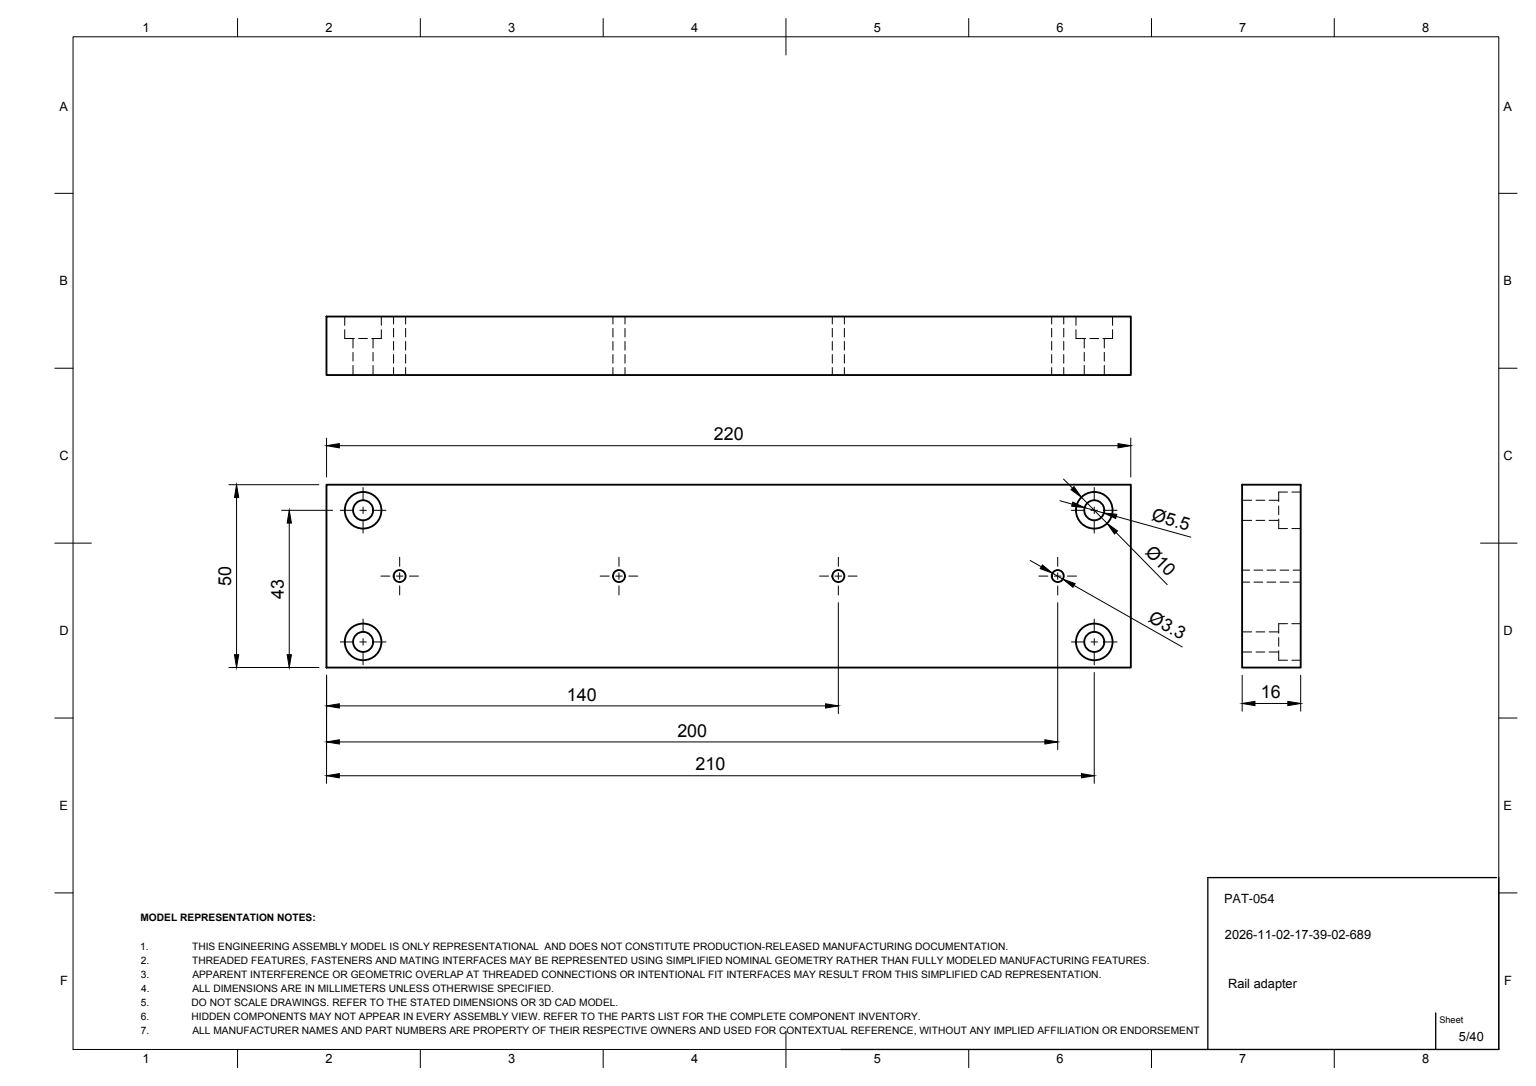
ISO-10303-21;
HEADER;
/* Generated by software containing ST-Developer
 * from STEP Tools, Inc. (www.steptools.com) 
 */

FILE_DESCRIPTION(
/* description */ ('PAT-054'),
/* implementation_level */ '2;1');

FILE_NAME(
/* name */ 'Rail adapter.step',
/* time_stamp */ '2026-10-29T16:38:13-07:00',
/* author */ (''),
/* organization */ (''),
/* preprocessor_version */ 'ST-DEVELOPER v20.2',
/* originating_system */ 'Autodesk Translation Framework v15.17.0.0',
/* authorisation */ '');

FILE_SCHEMA (('AUTOMOTIVE_DESIGN { 1 0 10303 214 3 1 1 }'));
ENDSEC;

DATA;
#10=MECHANICAL_DESIGN_GEOMETRIC_PRESENTATION_REPRESENTATION('',(#900),#33981);
#812=SHAPE_REPRESENTATION_RELATIONSHIP('SRR','None',#34185,#856);
#856=ADVANCED_BREP_SHAPE_REPRESENTATION('',(#959),#33933);
#900=STYLED_ITEM('',(#34510),#959);
#959=MANIFOLD_SOLID_BREP('Body1',#13011);
#1044=FACE_BOUND('',#2358,.T.);
#1045=FACE_BOUND('',#2361,.T.);
#1046=FACE_BOUND('',#2364,.T.);
#1047=FACE_BOUND('',#2367,.T.);
#1048=FACE_BOUND('',#2377,.T.);
#1049=FACE_BOUND('',#2378,.T.);
#1050=FACE_BOUND('',#2379,.T.);
#1051=FACE_BOUND('',#2380,.T.);
#1052=FACE_BOUND('',#2381,.T.);
#1053=FACE_BOUND('',#2382,.T.);
#1054=FACE_BOUND('',#2383,.T.);
#1055=FACE_BOUND('',#2384,.T.);
#1056=FACE_BOUND('',#2386,.T.);
#1057=FACE_BOUND('',#2387,.T.);
#1058=FACE_BOUND('',#2388,.T.);
#1059=FACE_BOUND('',#2389,.T.);
#1060=FACE_BOUND('',#2390,.T.);
#1061=FACE_BOUND('',#2391,.T.);
#1062=FACE_BOUND('',#2392,.T.);
#1063=FACE_BOUND('',#2393,.T.);
#1234=PLANE('',#13632);
#1235=PLANE('',#13637);
#1236=PLANE('',#13642);
#1237=PLANE('',#13647);
#1238=PLANE('',#13657);
#1239=PLANE('',#13658);
#1240=PLANE('',#13659);
#1241=PLANE('',#13660);
#1242=PLANE('',#13661);
#1243=PLANE('',#13662);
#1597=FACE_OUTER_BOUND('',#2352,.T.);
#1598=FACE_OUTER_BOUND('',#2353,.T.);
#1599=FACE_OUTER_BOUND('',#2354,.T.);
#1600=FACE_OUTER_BOUND('',#2355,.T.);
#1601=FACE_OUTER_BOUND('',#2356,.T.);
#1602=FACE_OUTER_BOUND('',#2357,.T.);
#1603=FACE_OUTER_BOUND('',#2359,.T.);
#1604=FACE_OUTER_BOUND('',#2360,.T.);
#1605=FACE_OUTER_BOUND('',#2362,.T.);
#1606=FACE_OUTER_BOUND('',#2363,.T.);
#1607=FACE_OUTER_BOUND('',#2365,.T.);
#1608=FACE_OUTER_BOUND('',#2366,.T.);
#1609=FACE_OUTER_BOUND('',#2368,.T.);
#1610=FACE_OUTER_BOUND('',#2369,.T.);
#1611=FACE_OUTER_BOUND('',#2370,.T.);
#1612=FACE_OUTER_BOUND('',#2371,.T.);
#1613=FACE_OUTER_BOUND('',#2372,.T.);
#1614=FACE_OUTER_BOUND('',#2373,.T.);
#1615=FACE_OUTER_BOUND('',#2374,.T.);
#1616=FACE_OUTER_BOUND('',#2375,.T.);
#1617=FACE_OUTER_BOUND('',#2376,.T.);
#1618=FACE_OUTER_BOUND('',#2385,.T.);
#2352=EDGE_LOOP('',(#8609,#8610,#8611,#8612));
#2353=EDGE_LOOP('',(#8613,#8614,#8615,#8616));
#2354=EDGE_LOOP('',(#8617,#8618,#8619,#8620));
#2355=EDGE_LOOP('',(#8621,#8622,#8623,#8624));
#2356=EDGE_LOOP('',(#8625,#8626,#8627,#8628));
#2357=EDGE_LOOP('',(#8629));
#2358=EDGE_LOOP('',(#8630));
#2359=EDGE_LOOP('',(#8631,#8632,#8633,#8634));
#2360=EDGE_LOOP('',(#8635));
#2361=EDGE_LOOP('',(#8636));
#2362=EDGE_LOOP('',(#8637,#8638,#8639,#8640));
#2363=EDGE_LOOP('',(#8641));
#2364=EDGE_LOOP('',(#8642));
#2365=EDGE_LOOP('',(#8643,#8644,#8645,#8646));
#2366=EDGE_LOOP('',(#8647));
#2367=EDGE_LOOP('',(#8648));
#2368=EDGE_LOOP('',(#8649,#8650,#8651,#8652));
#2369=EDGE_LOOP('',(#8653,#8654,#8655,#8656));
#2370=EDGE_LOOP('',(#8657,#8658,#8659,#8660));
#2371=EDGE_LOOP('',(#8661,#8662,#8663,#8664));
#2372=EDGE_LOOP('',(#8665,#8666,#8667,#8668));
#2373=EDGE_LOOP('',(#8669,#8670,#8671,#8672));
#2374=EDGE_LOOP('',(#8673,#8674,#8675,#8676));
#2375=EDGE_LOOP('',(#8677,#8678,#8679,#8680));
#2376=EDGE_LOOP('',(#8681,#8682,#8683,#8684));
#2377=EDGE_LOOP('',(#8685));
#2378=EDGE_LOOP('',(#8686));
#2379=EDGE_LOOP('',(#8687));
#2380=EDGE_LOOP('',(#8688));
#2381=EDGE_LOOP('',(#8689));
#2382=EDGE_LOOP('',(#8690));
#2383=EDGE_LOOP('',(#8691));
#2384=EDGE_LOOP('',(#8692));
#2385=EDGE_LOOP('',(#8693,#8694,#8695,#8696));
#2386=EDGE_LOOP('',(#8697));
#2387=EDGE_LOOP('',(#8698));
#2388=EDGE_LOOP('',(#8699));
#2389=EDGE_LOOP('',(#8700));
#2390=EDGE_LOOP('',(#8701));
#2391=EDGE_LOOP('',(#8702));
#2392=EDGE_LOOP('',(#8703));
#2393=EDGE_LOOP('',(#8704));
#3265=LINE('',#18616,#4199);
#3266=LINE('',#18622,#4200);
#3267=LINE('',#18628,#4201);
#3268=LINE('',#18634,#4202);
#3269=LINE('',#18640,#4203);
#3270=LINE('',#18649,#4204);
#3271=LINE('',#18658,#4205);
#3272=LINE('',#18667,#4206);
#3273=LINE('',#18675,#4207);
#3274=LINE('',#18679,#4208);
#3275=LINE('',#18683,#4209);
#3276=LINE('',#18687,#4210);
#3277=LINE('',#18691,#4211);
#3278=LINE('',#18693,#4212);
#3279=LINE('',#18695,#4213);
#3280=LINE('',#18696,#4214);
#3281=LINE('',#18699,#4215);
#3282=LINE('',#18701,#4216);
#3283=LINE('',#18702,#4217);
#3284=LINE('',#18705,#4218);
#3285=LINE('',#18707,#4219);
#3286=LINE('',#18708,#4220);
#3287=LINE('',#18710,#4221);
#3288=LINE('',#18711,#4222);
#4199=VECTOR('',#15038,0.164999999999999);
#4200=VECTOR('',#15045,0.164999999999999);
#4201=VECTOR('',#15052,0.165);
#4202=VECTOR('',#15059,0.164999999999999);
#4203=VECTOR('',#15066,0.5);
#4204=VECTOR('',#15077,0.5);
#4205=VECTOR('',#15088,0.5);
#4206=VECTOR('',#15099,0.5);
#4207=VECTOR('',#15110,0.274999999999999);
#4208=VECTOR('',#15115,0.275);
#4209=VECTOR('',#15120,0.275);
#4210=VECTOR('',#15125,0.274999999999999);
#4211=VECTOR('',#15128,1.);
#4212=VECTOR('',#15129,1.);
#4213=VECTOR('',#15130,1.);
#4214=VECTOR('',#15131,1.);
#4215=VECTOR('',#15134,1.);
#4216=VECTOR('',#15135,1.);
#4217=VECTOR('',#15136,1.);
#4218=VECTOR('',#15139,1.);
#4219=VECTOR('',#15140,1.);
#4220=VECTOR('',#15141,1.);
#4221=VECTOR('',#15144,1.);
#4222=VECTOR('',#15145,1.);
#5137=CIRCLE('',#13618,0.164999999999999);
#5138=CIRCLE('',#13619,0.164999999999999);
#5139=CIRCLE('',#13621,0.164999999999999);
#5140=CIRCLE('',#13622,0.164999999999999);
#5141=CIRCLE('',#13624,0.165);
#5142=CIRCLE('',#13625,0.165);
#5143=CIRCLE('',#13627,0.164999999999999);
#5144=CIRCLE('',#13628,0.164999999999999);
#5145=CIRCLE('',#13630,0.5);
#5146=CIRCLE('',#13631,0.5);
#5147=CIRCLE('',#13633,0.274999999999999);
#5148=CIRCLE('',#13635,0.5);
#5149=CIRCLE('',#13636,0.5);
#5150=CIRCLE('',#13638,0.275);
#5151=CIRCLE('',#13640,0.5);
#5152=CIRCLE('',#13641,0.5);
#5153=CIRCLE('',#13643,0.275);
#5154=CIRCLE('',#13645,0.5);
#5155=CIRCLE('',#13646,0.5);
#5156=CIRCLE('',#13648,0.274999999999999);
#5157=CIRCLE('',#13650,0.274999999999999);
#5158=CIRCLE('',#13652,0.275);
#5159=CIRCLE('',#13654,0.275);
#5160=CIRCLE('',#13656,0.274999999999999);
#5610=VERTEX_POINT('',#18613);
#5611=VERTEX_POINT('',#18615);
#5612=VERTEX_POINT('',#18619);
#5613=VERTEX_POINT('',#18621);
#5614=VERTEX_POINT('',#18625);
#5615=VERTEX_POINT('',#18627);
#5616=VERTEX_POINT('',#18631);
#5617=VERTEX_POINT('',#18633);
#5618=VERTEX_POINT('',#18637);
#5619=VERTEX_POINT('',#18639);
#5620=VERTEX_POINT('',#18643);
#5621=VERTEX_POINT('',#18646);
#5622=VERTEX_POINT('',#18648);
#5623=VERTEX_POINT('',#18652);
#5624=VERTEX_POINT('',#18655);
#5625=VERTEX_POINT('',#18657);
#5626=VERTEX_POINT('',#18661);
#5627=VERTEX_POINT('',#18664);
#5628=VERTEX_POINT('',#18666);
#5629=VERTEX_POINT('',#18670);
#5630=VERTEX_POINT('',#18673);
#5631=VERTEX_POINT('',#18677);
#5632=VERTEX_POINT('',#18681);
#5633=VERTEX_POINT('',#18685);
#5634=VERTEX_POINT('',#18689);
#5635=VERTEX_POINT('',#18690);
#5636=VERTEX_POINT('',#18692);
#5637=VERTEX_POINT('',#18694);
#5638=VERTEX_POINT('',#18698);
#5639=VERTEX_POINT('',#18700);
#5640=VERTEX_POINT('',#18704);
#5641=VERTEX_POINT('',#18706);
#6804=EDGE_CURVE('',#5610,#5610,#5137,.T.);
#6805=EDGE_CURVE('',#5610,#5611,#3265,.T.);
#6806=EDGE_CURVE('',#5611,#5611,#5138,.T.);
#6807=EDGE_CURVE('',#5612,#5612,#5139,.T.);
#6808=EDGE_CURVE('',#5612,#5613,#3266,.T.);
#6809=EDGE_CURVE('',#5613,#5613,#5140,.T.);
#6810=EDGE_CURVE('',#5614,#5614,#5141,.T.);
#6811=EDGE_CURVE('',#5614,#5615,#3267,.T.);
#6812=EDGE_CURVE('',#5615,#5615,#5142,.T.);
#6813=EDGE_CURVE('',#5616,#5616,#5143,.T.);
#6814=EDGE_CURVE('',#5616,#5617,#3268,.T.);
#6815=EDGE_CURVE('',#5617,#5617,#5144,.T.);
#6816=EDGE_CURVE('',#5618,#5618,#5145,.T.);
#6817=EDGE_CURVE('',#5618,#5619,#3269,.T.);
#6818=EDGE_CURVE('',#5619,#5619,#5146,.T.);
#6819=EDGE_CURVE('',#5620,#5620,#5147,.T.);
#6820=EDGE_CURVE('',#5621,#5621,#5148,.T.);
#6821=EDGE_CURVE('',#5621,#5622,#3270,.T.);
#6822=EDGE_CURVE('',#5622,#5622,#5149,.T.);
#6823=EDGE_CURVE('',#5623,#5623,#5150,.T.);
#6824=EDGE_CURVE('',#5624,#5624,#5151,.T.);
#6825=EDGE_CURVE('',#5624,#5625,#3271,.T.);
#6826=EDGE_CURVE('',#5625,#5625,#5152,.T.);
#6827=EDGE_CURVE('',#5626,#5626,#5153,.T.);
#6828=EDGE_CURVE('',#5627,#5627,#5154,.T.);
#6829=EDGE_CURVE('',#5627,#5628,#3272,.T.);
#6830=EDGE_CURVE('',#5628,#5628,#5155,.T.);
#6831=EDGE_CURVE('',#5629,#5629,#5156,.T.);
#6832=EDGE_CURVE('',#5630,#5630,#5157,.T.);
#6833=EDGE_CURVE('',#5630,#5620,#3273,.T.);
#6834=EDGE_CURVE('',#5631,#5631,#5158,.T.);
#6835=EDGE_CURVE('',#5631,#5623,#3274,.T.);
#6836=EDGE_CURVE('',#5632,#5632,#5159,.T.);
#6837=EDGE_CURVE('',#5632,#5626,#3275,.T.);
#6838=EDGE_CURVE('',#5633,#5633,#5160,.T.);
#6839=EDGE_CURVE('',#5633,#5629,#3276,.T.);
#6840=EDGE_CURVE('',#5634,#5635,#3277,.T.);
#6841=EDGE_CURVE('',#5635,#5636,#3278,.T.);
#6842=EDGE_CURVE('',#5637,#5636,#3279,.T.);
#6843=EDGE_CURVE('',#5634,#5637,#3280,.T.);
#6844=EDGE_CURVE('',#5638,#5634,#3281,.T.);
#6845=EDGE_CURVE('',#5639,#5637,#3282,.T.);
#6846=EDGE_CURVE('',#5638,#5639,#3283,.T.);
#6847=EDGE_CURVE('',#5640,#5638,#3284,.T.);
#6848=EDGE_CURVE('',#5641,#5639,#3285,.T.);
#6849=EDGE_CURVE('',#5640,#5641,#3286,.T.);
#6850=EDGE_CURVE('',#5635,#5640,#3287,.T.);
#6851=EDGE_CURVE('',#5636,#5641,#3288,.T.);
#8609=ORIENTED_EDGE('',*,*,#6804,.F.);
#8610=ORIENTED_EDGE('',*,*,#6805,.T.);
#8611=ORIENTED_EDGE('',*,*,#6806,.F.);
#8612=ORIENTED_EDGE('',*,*,#6805,.F.);
#8613=ORIENTED_EDGE('',*,*,#6807,.F.);
#8614=ORIENTED_EDGE('',*,*,#6808,.T.);
#8615=ORIENTED_EDGE('',*,*,#6809,.F.);
#8616=ORIENTED_EDGE('',*,*,#6808,.F.);
#8617=ORIENTED_EDGE('',*,*,#6810,.F.);
#8618=ORIENTED_EDGE('',*,*,#6811,.T.);
#8619=ORIENTED_EDGE('',*,*,#6812,.F.);
#8620=ORIENTED_EDGE('',*,*,#6811,.F.);
#8621=ORIENTED_EDGE('',*,*,#6813,.F.);
#8622=ORIENTED_EDGE('',*,*,#6814,.T.);
#8623=ORIENTED_EDGE('',*,*,#6815,.F.);
#8624=ORIENTED_EDGE('',*,*,#6814,.F.);
#8625=ORIENTED_EDGE('',*,*,#6816,.F.);
#8626=ORIENTED_EDGE('',*,*,#6817,.T.);
#8627=ORIENTED_EDGE('',*,*,#6818,.F.);
#8628=ORIENTED_EDGE('',*,*,#6817,.F.);
#8629=ORIENTED_EDGE('',*,*,#6816,.T.);
#8630=ORIENTED_EDGE('',*,*,#6819,.F.);
#8631=ORIENTED_EDGE('',*,*,#6820,.F.);
#8632=ORIENTED_EDGE('',*,*,#6821,.T.);
#8633=ORIENTED_EDGE('',*,*,#6822,.F.);
#8634=ORIENTED_EDGE('',*,*,#6821,.F.);
#8635=ORIENTED_EDGE('',*,*,#6820,.T.);
#8636=ORIENTED_EDGE('',*,*,#6823,.F.);
#8637=ORIENTED_EDGE('',*,*,#6824,.F.);
#8638=ORIENTED_EDGE('',*,*,#6825,.T.);
#8639=ORIENTED_EDGE('',*,*,#6826,.F.);
#8640=ORIENTED_EDGE('',*,*,#6825,.F.);
#8641=ORIENTED_EDGE('',*,*,#6824,.T.);
#8642=ORIENTED_EDGE('',*,*,#6827,.F.);
#8643=ORIENTED_EDGE('',*,*,#6828,.F.);
#8644=ORIENTED_EDGE('',*,*,#6829,.T.);
#8645=ORIENTED_EDGE('',*,*,#6830,.F.);
#8646=ORIENTED_EDGE('',*,*,#6829,.F.);
#8647=ORIENTED_EDGE('',*,*,#6828,.T.);
#8648=ORIENTED_EDGE('',*,*,#6831,.F.);
#8649=ORIENTED_EDGE('',*,*,#6832,.F.);
#8650=ORIENTED_EDGE('',*,*,#6833,.T.);
#8651=ORIENTED_EDGE('',*,*,#6819,.T.);
#8652=ORIENTED_EDGE('',*,*,#6833,.F.);
#8653=ORIENTED_EDGE('',*,*,#6834,.F.);
#8654=ORIENTED_EDGE('',*,*,#6835,.T.);
#8655=ORIENTED_EDGE('',*,*,#6823,.T.);
#8656=ORIENTED_EDGE('',*,*,#6835,.F.);
#8657=ORIENTED_EDGE('',*,*,#6836,.F.);
#8658=ORIENTED_EDGE('',*,*,#6837,.T.);
#8659=ORIENTED_EDGE('',*,*,#6827,.T.);
#8660=ORIENTED_EDGE('',*,*,#6837,.F.);
#8661=ORIENTED_EDGE('',*,*,#6838,.F.);
#8662=ORIENTED_EDGE('',*,*,#6839,.T.);
#8663=ORIENTED_EDGE('',*,*,#6831,.T.);
#8664=ORIENTED_EDGE('',*,*,#6839,.F.);
#8665=ORIENTED_EDGE('',*,*,#6840,.T.);
#8666=ORIENTED_EDGE('',*,*,#6841,.T.);
#8667=ORIENTED_EDGE('',*,*,#6842,.F.);
#8668=ORIENTED_EDGE('',*,*,#6843,.F.);
#8669=ORIENTED_EDGE('',*,*,#6844,.T.);
#8670=ORIENTED_EDGE('',*,*,#6843,.T.);
#8671=ORIENTED_EDGE('',*,*,#6845,.F.);
#8672=ORIENTED_EDGE('',*,*,#6846,.F.);
#8673=ORIENTED_EDGE('',*,*,#6847,.T.);
#8674=ORIENTED_EDGE('',*,*,#6846,.T.);
#8675=ORIENTED_EDGE('',*,*,#6848,.F.);
#8676=ORIENTED_EDGE('',*,*,#6849,.F.);
#8677=ORIENTED_EDGE('',*,*,#6850,.T.);
#8678=ORIENTED_EDGE('',*,*,#6849,.T.);
#8679=ORIENTED_EDGE('',*,*,#6851,.F.);
#8680=ORIENTED_EDGE('',*,*,#6841,.F.);
#8681=ORIENTED_EDGE('',*,*,#6851,.T.);
#8682=ORIENTED_EDGE('',*,*,#6848,.T.);
#8683=ORIENTED_EDGE('',*,*,#6845,.T.);
#8684=ORIENTED_EDGE('',*,*,#6842,.T.);
#8685=ORIENTED_EDGE('',*,*,#6818,.T.);
#8686=ORIENTED_EDGE('',*,*,#6822,.T.);
#8687=ORIENTED_EDGE('',*,*,#6826,.T.);
#8688=ORIENTED_EDGE('',*,*,#6830,.T.);
#8689=ORIENTED_EDGE('',*,*,#6815,.T.);
#8690=ORIENTED_EDGE('',*,*,#6812,.T.);
#8691=ORIENTED_EDGE('',*,*,#6809,.T.);
#8692=ORIENTED_EDGE('',*,*,#6806,.T.);
#8693=ORIENTED_EDGE('',*,*,#6850,.F.);
#8694=ORIENTED_EDGE('',*,*,#6840,.F.);
#8695=ORIENTED_EDGE('',*,*,#6844,.F.);
#8696=ORIENTED_EDGE('',*,*,#6847,.F.);
#8697=ORIENTED_EDGE('',*,*,#6838,.T.);
#8698=ORIENTED_EDGE('',*,*,#6836,.T.);
#8699=ORIENTED_EDGE('',*,*,#6834,.T.);
#8700=ORIENTED_EDGE('',*,*,#6832,.T.);
#8701=ORIENTED_EDGE('',*,*,#6813,.T.);
#8702=ORIENTED_EDGE('',*,*,#6810,.T.);
#8703=ORIENTED_EDGE('',*,*,#6807,.T.);
#8704=ORIENTED_EDGE('',*,*,#6804,.T.);
#11995=CYLINDRICAL_SURFACE('',#13617,0.164999999999999);
#11996=CYLINDRICAL_SURFACE('',#13620,0.164999999999999);
#11997=CYLINDRICAL_SURFACE('',#13623,0.165);
#11998=CYLINDRICAL_SURFACE('',#13626,0.164999999999999);
#11999=CYLINDRICAL_SURFACE('',#13629,0.5);
#12000=CYLINDRICAL_SURFACE('',#13634,0.5);
#12001=CYLINDRICAL_SURFACE('',#13639,0.5);
#12002=CYLINDRICAL_SURFACE('',#13644,0.5);
#12003=CYLINDRICAL_SURFACE('',#13649,0.274999999999999);
#12004=CYLINDRICAL_SURFACE('',#13651,0.275);
#12005=CYLINDRICAL_SURFACE('',#13653,0.275);
#12006=CYLINDRICAL_SURFACE('',#13655,0.274999999999999);
#12309=ADVANCED_FACE('',(#1597),#11995,.F.);
#12310=ADVANCED_FACE('',(#1598),#11996,.F.);
#12311=ADVANCED_FACE('',(#1599),#11997,.F.);
#12312=ADVANCED_FACE('',(#1600),#11998,.F.);
#12313=ADVANCED_FACE('',(#1601),#11999,.F.);
#12314=ADVANCED_FACE('',(#1602,#1044),#1234,.T.);
#12315=ADVANCED_FACE('',(#1603),#12000,.F.);
#12316=ADVANCED_FACE('',(#1604,#1045),#1235,.T.);
#12317=ADVANCED_FACE('',(#1605),#12001,.F.);
#12318=ADVANCED_FACE('',(#1606,#1046),#1236,.T.);
#12319=ADVANCED_FACE('',(#1607),#12002,.F.);
#12320=ADVANCED_FACE('',(#1608,#1047),#1237,.T.);
#12321=ADVANCED_FACE('',(#1609),#12003,.F.);
#12322=ADVANCED_FACE('',(#1610),#12004,.F.);
#12323=ADVANCED_FACE('',(#1611),#12005,.F.);
#12324=ADVANCED_FACE('',(#1612),#12006,.F.);
#12325=ADVANCED_FACE('',(#1613),#1238,.T.);
#12326=ADVANCED_FACE('',(#1614),#1239,.T.);
#12327=ADVANCED_FACE('',(#1615),#1240,.T.);
#12328=ADVANCED_FACE('',(#1616),#1241,.T.);
#12329=ADVANCED_FACE('',(#1617,#1048,#1049,#1050,#1051,#1052,#1053,#1054,
#1055),#1242,.T.);
#12330=ADVANCED_FACE('',(#1618,#1056,#1057,#1058,#1059,#1060,#1061,#1062,
#1063),#1243,.F.);
#13011=CLOSED_SHELL('',(#12309,#12310,#12311,#12312,#12313,#12314,#12315,
#12316,#12317,#12318,#12319,#12320,#12321,#12322,#12323,#12324,#12325,#12326,
#12327,#12328,#12329,#12330));
#13616=AXIS2_PLACEMENT_3D('',#18611,#15032,#15033);
#13617=AXIS2_PLACEMENT_3D('',#18612,#15034,#15035);
#13618=AXIS2_PLACEMENT_3D('',#18614,#15036,#15037);
#13619=AXIS2_PLACEMENT_3D('',#18617,#15039,#15040);
#13620=AXIS2_PLACEMENT_3D('',#18618,#15041,#15042);
#13621=AXIS2_PLACEMENT_3D('',#18620,#15043,#15044);
#13622=AXIS2_PLACEMENT_3D('',#18623,#15046,#15047);
#13623=AXIS2_PLACEMENT_3D('',#18624,#15048,#15049);
#13624=AXIS2_PLACEMENT_3D('',#18626,#15050,#15051);
#13625=AXIS2_PLACEMENT_3D('',#18629,#15053,#15054);
#13626=AXIS2_PLACEMENT_3D('',#18630,#15055,#15056);
#13627=AXIS2_PLACEMENT_3D('',#18632,#15057,#15058);
#13628=AXIS2_PLACEMENT_3D('',#18635,#15060,#15061);
#13629=AXIS2_PLACEMENT_3D('',#18636,#15062,#15063);
#13630=AXIS2_PLACEMENT_3D('',#18638,#15064,#15065);
#13631=AXIS2_PLACEMENT_3D('',#18641,#15067,#15068);
#13632=AXIS2_PLACEMENT_3D('',#18642,#15069,#15070);
#13633=AXIS2_PLACEMENT_3D('',#18644,#15071,#15072);
#13634=AXIS2_PLACEMENT_3D('',#18645,#15073,#15074);
#13635=AXIS2_PLACEMENT_3D('',#18647,#15075,#15076);
#13636=AXIS2_PLACEMENT_3D('',#18650,#15078,#15079);
#13637=AXIS2_PLACEMENT_3D('',#18651,#15080,#15081);
#13638=AXIS2_PLACEMENT_3D('',#18653,#15082,#15083);
#13639=AXIS2_PLACEMENT_3D('',#18654,#15084,#15085);
#13640=AXIS2_PLACEMENT_3D('',#18656,#15086,#15087);
#13641=AXIS2_PLACEMENT_3D('',#18659,#15089,#15090);
#13642=AXIS2_PLACEMENT_3D('',#18660,#15091,#15092);
#13643=AXIS2_PLACEMENT_3D('',#18662,#15093,#15094);
#13644=AXIS2_PLACEMENT_3D('',#18663,#15095,#15096);
#13645=AXIS2_PLACEMENT_3D('',#18665,#15097,#15098);
#13646=AXIS2_PLACEMENT_3D('',#18668,#15100,#15101);
#13647=AXIS2_PLACEMENT_3D('',#18669,#15102,#15103);
#13648=AXIS2_PLACEMENT_3D('',#18671,#15104,#15105);
#13649=AXIS2_PLACEMENT_3D('',#18672,#15106,#15107);
#13650=AXIS2_PLACEMENT_3D('',#18674,#15108,#15109);
#13651=AXIS2_PLACEMENT_3D('',#18676,#15111,#15112);
#13652=AXIS2_PLACEMENT_3D('',#18678,#15113,#15114);
#13653=AXIS2_PLACEMENT_3D('',#18680,#15116,#15117);
#13654=AXIS2_PLACEMENT_3D('',#18682,#15118,#15119);
#13655=AXIS2_PLACEMENT_3D('',#18684,#15121,#15122);
#13656=AXIS2_PLACEMENT_3D('',#18686,#15123,#15124);
#13657=AXIS2_PLACEMENT_3D('',#18688,#15126,#15127);
#13658=AXIS2_PLACEMENT_3D('',#18697,#15132,#15133);
#13659=AXIS2_PLACEMENT_3D('',#18703,#15137,#15138);
#13660=AXIS2_PLACEMENT_3D('',#18709,#15142,#15143);
#13661=AXIS2_PLACEMENT_3D('',#18712,#15146,#15147);
#13662=AXIS2_PLACEMENT_3D('',#18713,#15148,#15149);
#15032=DIRECTION('axis',(0.,0.,1.));
#15033=DIRECTION('refdir',(1.,0.,0.));
#15034=DIRECTION('center_axis',(0.,0.,1.));
#15035=DIRECTION('ref_axis',(1.,0.,0.));
#15036=DIRECTION('center_axis',(0.,0.,1.));
#15037=DIRECTION('ref_axis',(1.,0.,0.));
#15038=DIRECTION('',(0.,0.,1.));
#15039=DIRECTION('center_axis',(0.,0.,-1.));
#15040=DIRECTION('ref_axis',(1.,0.,0.));
#15041=DIRECTION('center_axis',(0.,0.,1.));
#15042=DIRECTION('ref_axis',(1.,0.,0.));
#15043=DIRECTION('center_axis',(0.,0.,1.));
#15044=DIRECTION('ref_axis',(1.,0.,0.));
#15045=DIRECTION('',(0.,0.,1.));
#15046=DIRECTION('center_axis',(0.,0.,-1.));
#15047=DIRECTION('ref_axis',(1.,0.,0.));
#15048=DIRECTION('center_axis',(0.,0.,1.));
#15049=DIRECTION('ref_axis',(1.,0.,0.));
#15050=DIRECTION('center_axis',(0.,0.,1.));
#15051=DIRECTION('ref_axis',(1.,0.,0.));
#15052=DIRECTION('',(0.,0.,1.));
#15053=DIRECTION('center_axis',(0.,0.,-1.));
#15054=DIRECTION('ref_axis',(1.,0.,0.));
#15055=DIRECTION('center_axis',(0.,0.,1.));
#15056=DIRECTION('ref_axis',(1.,0.,0.));
#15057=DIRECTION('center_axis',(0.,0.,1.));
#15058=DIRECTION('ref_axis',(1.,0.,0.));
#15059=DIRECTION('',(0.,0.,1.));
#15060=DIRECTION('center_axis',(0.,0.,-1.));
#15061=DIRECTION('ref_axis',(1.,0.,0.));
#15062=DIRECTION('center_axis',(0.,0.,1.));
#15063=DIRECTION('ref_axis',(1.,0.,0.));
#15064=DIRECTION('center_axis',(0.,0.,1.));
#15065=DIRECTION('ref_axis',(1.,0.,0.));
#15066=DIRECTION('',(0.,0.,1.));
#15067=DIRECTION('center_axis',(0.,0.,-1.));
#15068=DIRECTION('ref_axis',(1.,0.,0.));
#15069=DIRECTION('center_axis',(0.,0.,1.));
#15070=DIRECTION('ref_axis',(1.,0.,0.));
#15071=DIRECTION('center_axis',(0.,0.,1.));
#15072=DIRECTION('ref_axis',(1.,0.,0.));
#15073=DIRECTION('center_axis',(0.,0.,1.));
#15074=DIRECTION('ref_axis',(1.,0.,0.));
#15075=DIRECTION('center_axis',(0.,0.,1.));
#15076=DIRECTION('ref_axis',(1.,0.,0.));
#15077=DIRECTION('',(0.,0.,1.));
#15078=DIRECTION('center_axis',(0.,0.,-1.));
#15079=DIRECTION('ref_axis',(1.,0.,0.));
#15080=DIRECTION('center_axis',(0.,0.,1.));
#15081=DIRECTION('ref_axis',(1.,0.,0.));
#15082=DIRECTION('center_axis',(0.,0.,1.));
#15083=DIRECTION('ref_axis',(1.,0.,0.));
#15084=DIRECTION('center_axis',(0.,0.,1.));
#15085=DIRECTION('ref_axis',(1.,0.,0.));
#15086=DIRECTION('center_axis',(0.,0.,1.));
#15087=DIRECTION('ref_axis',(1.,0.,0.));
#15088=DIRECTION('',(0.,0.,1.));
#15089=DIRECTION('center_axis',(0.,0.,-1.));
#15090=DIRECTION('ref_axis',(1.,0.,0.));
#15091=DIRECTION('center_axis',(0.,0.,1.));
#15092=DIRECTION('ref_axis',(1.,0.,0.));
#15093=DIRECTION('center_axis',(0.,0.,1.));
#15094=DIRECTION('ref_axis',(1.,0.,0.));
#15095=DIRECTION('center_axis',(0.,0.,1.));
#15096=DIRECTION('ref_axis',(1.,0.,0.));
#15097=DIRECTION('center_axis',(0.,0.,1.));
#15098=DIRECTION('ref_axis',(1.,0.,0.));
#15099=DIRECTION('',(0.,0.,1.));
#15100=DIRECTION('center_axis',(0.,0.,-1.));
#15101=DIRECTION('ref_axis',(1.,0.,0.));
#15102=DIRECTION('center_axis',(0.,0.,1.));
#15103=DIRECTION('ref_axis',(1.,0.,0.));
#15104=DIRECTION('center_axis',(0.,0.,1.));
#15105=DIRECTION('ref_axis',(1.,0.,0.));
#15106=DIRECTION('center_axis',(0.,0.,1.));
#15107=DIRECTION('ref_axis',(1.,0.,0.));
#15108=DIRECTION('center_axis',(0.,0.,1.));
#15109=DIRECTION('ref_axis',(1.,0.,0.));
#15110=DIRECTION('',(0.,0.,1.));
#15111=DIRECTION('center_axis',(0.,0.,1.));
#15112=DIRECTION('ref_axis',(1.,0.,0.));
#15113=DIRECTION('center_axis',(0.,0.,1.));
#15114=DIRECTION('ref_axis',(1.,0.,0.));
#15115=DIRECTION('',(0.,0.,1.));
#15116=DIRECTION('center_axis',(0.,0.,1.));
#15117=DIRECTION('ref_axis',(1.,0.,0.));
#15118=DIRECTION('center_axis',(0.,0.,1.));
#15119=DIRECTION('ref_axis',(1.,0.,0.));
#15120=DIRECTION('',(0.,0.,1.));
#15121=DIRECTION('center_axis',(0.,0.,1.));
#15122=DIRECTION('ref_axis',(1.,0.,0.));
#15123=DIRECTION('center_axis',(0.,0.,1.));
#15124=DIRECTION('ref_axis',(1.,0.,0.));
#15125=DIRECTION('',(0.,0.,1.));
#15126=DIRECTION('center_axis',(0.,1.,0.));
#15127=DIRECTION('ref_axis',(-1.,0.,0.));
#15128=DIRECTION('',(-1.,0.,0.));
#15129=DIRECTION('',(0.,0.,1.));
#15130=DIRECTION('',(-1.,0.,0.));
#15131=DIRECTION('',(0.,0.,1.));
#15132=DIRECTION('center_axis',(1.,0.,0.));
#15133=DIRECTION('ref_axis',(0.,1.,0.));
#15134=DIRECTION('',(0.,1.,0.));
#15135=DIRECTION('',(0.,1.,0.));
#15136=DIRECTION('',(0.,0.,1.));
#15137=DIRECTION('center_axis',(0.,-1.,0.));
#15138=DIRECTION('ref_axis',(1.,0.,0.));
#15139=DIRECTION('',(1.,0.,0.));
#15140=DIRECTION('',(1.,0.,0.));
#15141=DIRECTION('',(0.,0.,1.));
#15142=DIRECTION('center_axis',(-1.,0.,0.));
#15143=DIRECTION('ref_axis',(0.,-1.,0.));
#15144=DIRECTION('',(0.,-1.,0.));
#15145=DIRECTION('',(0.,-1.,0.));
#15146=DIRECTION('center_axis',(0.,0.,1.));
#15147=DIRECTION('ref_axis',(1.,0.,0.));
#15148=DIRECTION('center_axis',(0.,0.,1.));
#15149=DIRECTION('ref_axis',(1.,0.,0.));
#18611=CARTESIAN_POINT('',(0.,0.,0.));
#18612=CARTESIAN_POINT('Origin',(14.,-6.,1.1));
#18613=CARTESIAN_POINT('',(13.835,-6.,1.2));
#18614=CARTESIAN_POINT('Origin',(14.,-6.,1.2));
#18615=CARTESIAN_POINT('',(13.835,-6.,2.8));
#18616=CARTESIAN_POINT('',(13.835,-6.,1.1));
#18617=CARTESIAN_POINT('Origin',(14.,-6.,2.8));
#18618=CARTESIAN_POINT('Origin',(8.,-6.,1.1));
#18619=CARTESIAN_POINT('',(7.835,-6.,1.2));
#18620=CARTESIAN_POINT('Origin',(8.,-6.,1.2));
#18621=CARTESIAN_POINT('',(7.835,-6.,2.8));
#18622=CARTESIAN_POINT('',(7.835,-6.,1.1));
#18623=CARTESIAN_POINT('Origin',(8.,-6.,2.8));
#18624=CARTESIAN_POINT('Origin',(2.,-6.,1.1));
#18625=CARTESIAN_POINT('',(1.835,-6.,1.2));
#18626=CARTESIAN_POINT('Origin',(2.,-6.,1.2));
#18627=CARTESIAN_POINT('',(1.835,-6.,2.8));
#18628=CARTESIAN_POINT('',(1.835,-6.,1.1));
#18629=CARTESIAN_POINT('Origin',(2.,-6.,2.8));
#18630=CARTESIAN_POINT('Origin',(20.,-6.,1.1));
#18631=CARTESIAN_POINT('',(19.835,-6.,1.2));
#18632=CARTESIAN_POINT('Origin',(20.,-6.,1.2));
#18633=CARTESIAN_POINT('',(19.835,-6.,2.8));
#18634=CARTESIAN_POINT('',(19.835,-6.,1.1));
#18635=CARTESIAN_POINT('Origin',(20.,-6.,2.8));
#18636=CARTESIAN_POINT('Origin',(21.,-7.8,2.2));
#18637=CARTESIAN_POINT('',(20.5,-7.8,2.2));
#18638=CARTESIAN_POINT('Origin',(21.,-7.8,2.2));
#18639=CARTESIAN_POINT('',(20.5,-7.8,2.8));
#18640=CARTESIAN_POINT('',(20.5,-7.8,2.2));
#18641=CARTESIAN_POINT('Origin',(21.,-7.8,2.8));
#18642=CARTESIAN_POINT('Origin',(21.,-7.8,2.2));
#18643=CARTESIAN_POINT('',(20.725,-7.8,2.2));
#18644=CARTESIAN_POINT('Origin',(21.,-7.8,2.2));
#18645=CARTESIAN_POINT('Origin',(1.,-4.2,2.2));
#18646=CARTESIAN_POINT('',(0.5,-4.2,2.2));
#18647=CARTESIAN_POINT('Origin',(1.,-4.2,2.2));
#18648=CARTESIAN_POINT('',(0.5,-4.2,2.8));
#18649=CARTESIAN_POINT('',(0.5,-4.2,2.2));
#18650=CARTESIAN_POINT('Origin',(1.,-4.2,2.8));
#18651=CARTESIAN_POINT('Origin',(1.,-4.2,2.2));
#18652=CARTESIAN_POINT('',(0.725,-4.2,2.2));
#18653=CARTESIAN_POINT('Origin',(1.,-4.2,2.2));
#18654=CARTESIAN_POINT('Origin',(1.,-7.8,2.2));
#18655=CARTESIAN_POINT('',(0.5,-7.8,2.2));
#18656=CARTESIAN_POINT('Origin',(1.,-7.8,2.2));
#18657=CARTESIAN_POINT('',(0.5,-7.8,2.8));
#18658=CARTESIAN_POINT('',(0.5,-7.8,2.2));
#18659=CARTESIAN_POINT('Origin',(1.,-7.8,2.8));
#18660=CARTESIAN_POINT('Origin',(1.,-7.8,2.2));
#18661=CARTESIAN_POINT('',(0.725,-7.8,2.2));
#18662=CARTESIAN_POINT('Origin',(1.,-7.8,2.2));
#18663=CARTESIAN_POINT('Origin',(21.,-4.2,2.2));
#18664=CARTESIAN_POINT('',(20.5,-4.2,2.2));
#18665=CARTESIAN_POINT('Origin',(21.,-4.2,2.2));
#18666=CARTESIAN_POINT('',(20.5,-4.2,2.8));
#18667=CARTESIAN_POINT('',(20.5,-4.2,2.2));
#18668=CARTESIAN_POINT('Origin',(21.,-4.2,2.8));
#18669=CARTESIAN_POINT('Origin',(21.,-4.2,2.2));
#18670=CARTESIAN_POINT('',(20.725,-4.2,2.2));
#18671=CARTESIAN_POINT('Origin',(21.,-4.2,2.2));
#18672=CARTESIAN_POINT('Origin',(21.,-7.8,1.1));
#18673=CARTESIAN_POINT('',(20.725,-7.8,1.2));
#18674=CARTESIAN_POINT('Origin',(21.,-7.8,1.2));
#18675=CARTESIAN_POINT('',(20.725,-7.8,1.1));
#18676=CARTESIAN_POINT('Origin',(1.,-4.2,1.1));
#18677=CARTESIAN_POINT('',(0.725,-4.2,1.2));
#18678=CARTESIAN_POINT('Origin',(1.,-4.2,1.2));
#18679=CARTESIAN_POINT('',(0.725,-4.2,1.1));
#18680=CARTESIAN_POINT('Origin',(1.,-7.8,1.1));
#18681=CARTESIAN_POINT('',(0.725,-7.8,1.2));
#18682=CARTESIAN_POINT('Origin',(1.,-7.8,1.2));
#18683=CARTESIAN_POINT('',(0.725,-7.8,1.1));
#18684=CARTESIAN_POINT('Origin',(21.,-4.2,1.1));
#18685=CARTESIAN_POINT('',(20.725,-4.2,1.2));
#18686=CARTESIAN_POINT('Origin',(21.,-4.2,1.2));
#18687=CARTESIAN_POINT('',(20.725,-4.2,1.1));
#18688=CARTESIAN_POINT('Origin',(22.,-3.5,1.2));
#18689=CARTESIAN_POINT('',(22.,-3.5,1.2));
#18690=CARTESIAN_POINT('',(0.,-3.5,1.2));
#18691=CARTESIAN_POINT('',(22.,-3.5,1.2));
#18692=CARTESIAN_POINT('',(0.,-3.5,2.8));
#18693=CARTESIAN_POINT('',(0.,-3.5,1.2));
#18694=CARTESIAN_POINT('',(22.,-3.5,2.8));
#18695=CARTESIAN_POINT('',(22.,-3.5,2.8));
#18696=CARTESIAN_POINT('',(22.,-3.5,1.2));
#18697=CARTESIAN_POINT('Origin',(22.,-8.5,1.2));
#18698=CARTESIAN_POINT('',(22.,-8.5,1.2));
#18699=CARTESIAN_POINT('',(22.,-8.5,1.2));
#18700=CARTESIAN_POINT('',(22.,-8.5,2.8));
#18701=CARTESIAN_POINT('',(22.,-8.5,2.8));
#18702=CARTESIAN_POINT('',(22.,-8.5,1.2));
#18703=CARTESIAN_POINT('Origin',(0.,-8.5,1.2));
#18704=CARTESIAN_POINT('',(0.,-8.5,1.2));
#18705=CARTESIAN_POINT('',(0.,-8.5,1.2));
#18706=CARTESIAN_POINT('',(0.,-8.5,2.8));
#18707=CARTESIAN_POINT('',(0.,-8.5,2.8));
#18708=CARTESIAN_POINT('',(0.,-8.5,1.2));
#18709=CARTESIAN_POINT('Origin',(0.,-3.5,1.2));
#18710=CARTESIAN_POINT('',(0.,-3.5,1.2));
#18711=CARTESIAN_POINT('',(0.,-3.5,2.8));
#18712=CARTESIAN_POINT('Origin',(11.,-6.,2.8));
#18713=CARTESIAN_POINT('Origin',(11.,-6.,1.2));
#33881=UNCERTAINTY_MEASURE_WITH_UNIT(LENGTH_MEASURE(0.001),#33982,
'DISTANCE_ACCURACY_VALUE',
'Maximum model space distance between geometric entities at asserted c
onnectivities');
#33929=UNCERTAINTY_MEASURE_WITH_UNIT(LENGTH_MEASURE(0.001),#33982,
'DISTANCE_ACCURACY_VALUE',
'Maximum model space distance between geometric entities at asserted c
onnectivities');
#33933=(
GEOMETRIC_REPRESENTATION_CONTEXT(3)
GLOBAL_UNCERTAINTY_ASSIGNED_CONTEXT((#33881))
GLOBAL_UNIT_ASSIGNED_CONTEXT((#33982,#33984,#33985))
REPRESENTATION_CONTEXT('','3D')
);
#33981=(
GEOMETRIC_REPRESENTATION_CONTEXT(3)
GLOBAL_UNCERTAINTY_ASSIGNED_CONTEXT((#33929))
GLOBAL_UNIT_ASSIGNED_CONTEXT((#33982,#33984,#33985))
REPRESENTATION_CONTEXT('','3D')
);
#33982=(
LENGTH_UNIT()
NAMED_UNIT(*)
SI_UNIT(.CENTI.,.METRE.)
);
#33984=(
NAMED_UNIT(*)
PLANE_ANGLE_UNIT()
SI_UNIT($,.RADIAN.)
);
#33985=(
NAMED_UNIT(*)
SI_UNIT($,.STERADIAN.)
SOLID_ANGLE_UNIT()
);
#33989=SHAPE_DEFINITION_REPRESENTATION(#34040,#34185);
#34040=PRODUCT_DEFINITION_SHAPE('',$,#34237);
#34185=SHAPE_REPRESENTATION('',(#13616),#33933);
#34233=PRODUCT_DEFINITION_CONTEXT('part definition',#34388,'design');
#34237=PRODUCT_DEFINITION('Rail adapter','Rail adapter',#34288,#34233);
#34288=PRODUCT_DEFINITION_FORMATION('',$,#34393);
#34388=APPLICATION_CONTEXT(
'Core Data for Automotive Mechanical Design Process');
#34389=PRODUCT_CONTEXT('part definition',#34388,'mechanical');
#34393=PRODUCT('Rail adapter','Rail adapter','Rail adapter',(#34389));
#34504=COLOUR_RGB('Sky Blue',0.24,0.69,0.87);
#34505=FILL_AREA_STYLE_COLOUR('',#34504);
#34506=FILL_AREA_STYLE('',(#34505));
#34507=SURFACE_STYLE_FILL_AREA(#34506);
#34508=SURFACE_SIDE_STYLE('',(#34507));
#34509=SURFACE_STYLE_USAGE(.BOTH.,#34508);
#34510=PRESENTATION_STYLE_ASSIGNMENT((#34509));
ENDSEC;
END-ISO-10303-21;
